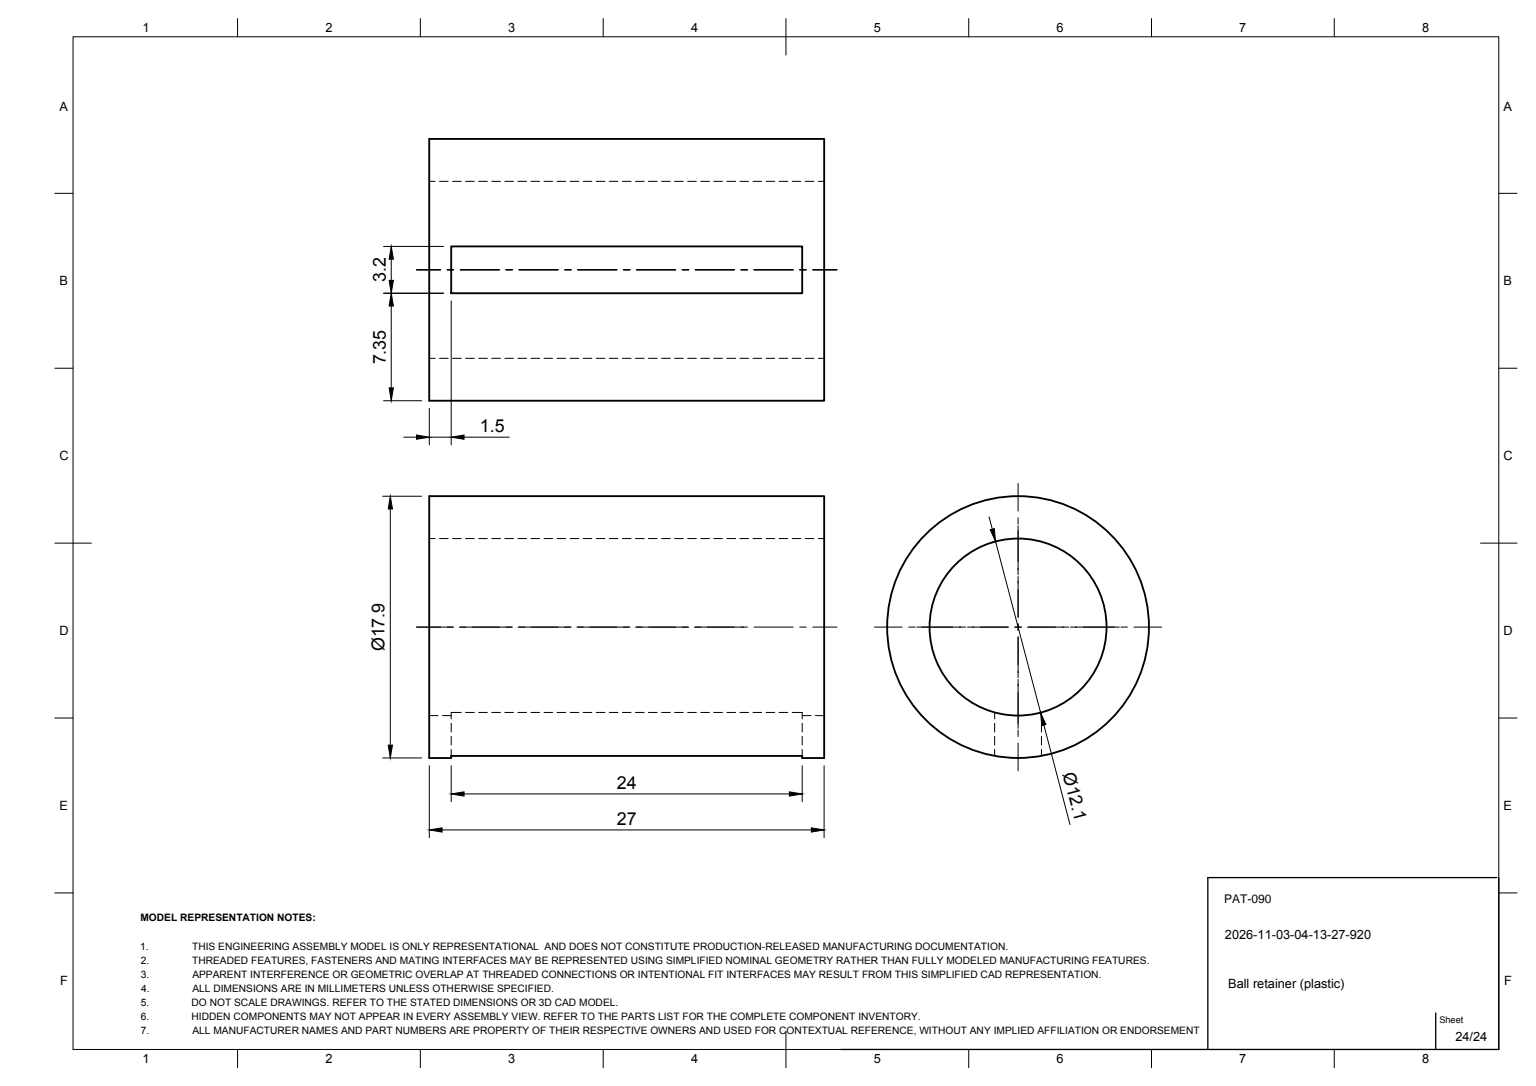
ISO-10303-21;
HEADER;
/* Generated by software containing ST-Developer
 * from STEP Tools, Inc. (www.steptools.com) 
 */

FILE_DESCRIPTION(
/* description */ ('Round-Shaft Linear Stage with Ball Bushings'),
/* implementation_level */ '2;1');

FILE_NAME(
/* name */ 'Ball retainer (plastic).step',
/* time_stamp */ '2026-10-27T10:47:55-07:00',
/* author */ (''),
/* organization */ (''),
/* preprocessor_version */ 'ST-DEVELOPER v20.2',
/* originating_system */ 'Autodesk Translation Framework v15.17.0.0',
/* authorisation */ '');

FILE_SCHEMA (('AUTOMOTIVE_DESIGN { 1 0 10303 214 3 1 1 }'));
ENDSEC;

DATA;
#10=MECHANICAL_DESIGN_GEOMETRIC_PRESENTATION_REPRESENTATION('',(#318),#7835);
#276=SHAPE_REPRESENTATION_RELATIONSHIP('SRR','None',#7966,#297);
#297=ADVANCED_BREP_SHAPE_REPRESENTATION('',(#338),#7830);
#318=STYLED_ITEM('',(#8137),#338);
#338=MANIFOLD_SOLID_BREP('Body1',#4409);
#450=FACE_BOUND('',#1182,.T.);
#451=FACE_BOUND('',#1184,.T.);
#452=FACE_BOUND('',#1186,.T.);
#453=FACE_BOUND('',#1188,.T.);
#575=PLANE('',#5017);
#576=PLANE('',#5020);
#577=PLANE('',#5021);
#578=PLANE('',#5024);
#579=PLANE('',#5025);
#580=PLANE('',#5030);
#810=FACE_OUTER_BOUND('',#1177,.T.);
#811=FACE_OUTER_BOUND('',#1178,.T.);
#812=FACE_OUTER_BOUND('',#1179,.T.);
#813=FACE_OUTER_BOUND('',#1180,.T.);
#814=FACE_OUTER_BOUND('',#1181,.T.);
#815=FACE_OUTER_BOUND('',#1183,.T.);
#816=FACE_OUTER_BOUND('',#1185,.T.);
#817=FACE_OUTER_BOUND('',#1187,.T.);
#1177=EDGE_LOOP('',(#3812,#3813,#3814,#3815));
#1178=EDGE_LOOP('',(#3816,#3817,#3818,#3819));
#1179=EDGE_LOOP('',(#3820,#3821,#3822,#3823));
#1180=EDGE_LOOP('',(#3824,#3825,#3826,#3827));
#1181=EDGE_LOOP('',(#3828));
#1182=EDGE_LOOP('',(#3829));
#1183=EDGE_LOOP('',(#3830,#3831,#3832,#3833));
#1184=EDGE_LOOP('',(#3834,#3835,#3836,#3837));
#1185=EDGE_LOOP('',(#3838));
#1186=EDGE_LOOP('',(#3839));
#1187=EDGE_LOOP('',(#3840,#3841,#3842,#3843));
#1188=EDGE_LOOP('',(#3844,#3845,#3846,#3847));
#1505=LINE('',#7470,#1845);
#1506=LINE('',#7473,#1846);
#1507=LINE('',#7476,#1847);
#1508=LINE('',#7478,#1848);
#1509=LINE('',#7479,#1849);
#1510=LINE('',#7485,#1850);
#1511=LINE('',#7487,#1851);
#1512=LINE('',#7488,#1852);
#1513=LINE('',#7497,#1853);
#1514=LINE('',#7502,#1854);
#1845=VECTOR('',#6172,1.);
#1846=VECTOR('',#6175,1.);
#1847=VECTOR('',#6178,1.);
#1848=VECTOR('',#6179,1.);
#1849=VECTOR('',#6180,1.);
#1850=VECTOR('',#6187,1.);
#1851=VECTOR('',#6190,1.);
#1852=VECTOR('',#6191,1.);
#1853=VECTOR('',#6202,0.895);
#1854=VECTOR('',#6209,0.605);
#2082=CIRCLE('',#5018,0.895);
#2083=CIRCLE('',#5019,0.605);
#2084=CIRCLE('',#5022,0.895);
#2085=CIRCLE('',#5023,0.605);
#2086=CIRCLE('',#5026,0.895);
#2087=CIRCLE('',#5027,0.605);
#2088=CIRCLE('',#5029,0.895);
#2089=CIRCLE('',#5031,0.605);
#2389=VERTEX_POINT('',#7466);
#2390=VERTEX_POINT('',#7467);
#2391=VERTEX_POINT('',#7469);
#2392=VERTEX_POINT('',#7471);
#2393=VERTEX_POINT('',#7475);
#2394=VERTEX_POINT('',#7477);
#2395=VERTEX_POINT('',#7481);
#2396=VERTEX_POINT('',#7483);
#2397=VERTEX_POINT('',#7490);
#2398=VERTEX_POINT('',#7492);
#2399=VERTEX_POINT('',#7495);
#2400=VERTEX_POINT('',#7499);
#2874=EDGE_CURVE('',#2389,#2390,#2082,.T.);
#2875=EDGE_CURVE('',#2391,#2389,#1505,.T.);
#2876=EDGE_CURVE('',#2392,#2391,#2083,.T.);
#2877=EDGE_CURVE('',#2390,#2392,#1506,.T.);
#2878=EDGE_CURVE('',#2390,#2393,#1507,.T.);
#2879=EDGE_CURVE('',#2394,#2392,#1508,.T.);
#2880=EDGE_CURVE('',#2394,#2393,#1509,.T.);
#2881=EDGE_CURVE('',#2393,#2395,#2084,.T.);
#2882=EDGE_CURVE('',#2396,#2394,#2085,.T.);
#2883=EDGE_CURVE('',#2395,#2396,#1510,.T.);
#2884=EDGE_CURVE('',#2395,#2389,#1511,.T.);
#2885=EDGE_CURVE('',#2391,#2396,#1512,.T.);
#2886=EDGE_CURVE('',#2397,#2397,#2086,.T.);
#2887=EDGE_CURVE('',#2398,#2398,#2087,.T.);
#2888=EDGE_CURVE('',#2399,#2399,#2088,.T.);
#2889=EDGE_CURVE('',#2399,#2397,#1513,.T.);
#2890=EDGE_CURVE('',#2400,#2400,#2089,.T.);
#2891=EDGE_CURVE('',#2400,#2398,#1514,.T.);
#3812=ORIENTED_EDGE('',*,*,#2874,.F.);
#3813=ORIENTED_EDGE('',*,*,#2875,.F.);
#3814=ORIENTED_EDGE('',*,*,#2876,.F.);
#3815=ORIENTED_EDGE('',*,*,#2877,.F.);
#3816=ORIENTED_EDGE('',*,*,#2878,.F.);
#3817=ORIENTED_EDGE('',*,*,#2877,.T.);
#3818=ORIENTED_EDGE('',*,*,#2879,.F.);
#3819=ORIENTED_EDGE('',*,*,#2880,.T.);
#3820=ORIENTED_EDGE('',*,*,#2881,.F.);
#3821=ORIENTED_EDGE('',*,*,#2880,.F.);
#3822=ORIENTED_EDGE('',*,*,#2882,.F.);
#3823=ORIENTED_EDGE('',*,*,#2883,.F.);
#3824=ORIENTED_EDGE('',*,*,#2884,.F.);
#3825=ORIENTED_EDGE('',*,*,#2883,.T.);
#3826=ORIENTED_EDGE('',*,*,#2885,.F.);
#3827=ORIENTED_EDGE('',*,*,#2875,.T.);
#3828=ORIENTED_EDGE('',*,*,#2886,.F.);
#3829=ORIENTED_EDGE('',*,*,#2887,.T.);
#3830=ORIENTED_EDGE('',*,*,#2888,.F.);
#3831=ORIENTED_EDGE('',*,*,#2889,.T.);
#3832=ORIENTED_EDGE('',*,*,#2886,.T.);
#3833=ORIENTED_EDGE('',*,*,#2889,.F.);
#3834=ORIENTED_EDGE('',*,*,#2881,.T.);
#3835=ORIENTED_EDGE('',*,*,#2884,.T.);
#3836=ORIENTED_EDGE('',*,*,#2874,.T.);
#3837=ORIENTED_EDGE('',*,*,#2878,.T.);
#3838=ORIENTED_EDGE('',*,*,#2888,.T.);
#3839=ORIENTED_EDGE('',*,*,#2890,.F.);
#3840=ORIENTED_EDGE('',*,*,#2890,.T.);
#3841=ORIENTED_EDGE('',*,*,#2891,.T.);
#3842=ORIENTED_EDGE('',*,*,#2887,.F.);
#3843=ORIENTED_EDGE('',*,*,#2891,.F.);
#3844=ORIENTED_EDGE('',*,*,#2882,.T.);
#3845=ORIENTED_EDGE('',*,*,#2879,.T.);
#3846=ORIENTED_EDGE('',*,*,#2876,.T.);
#3847=ORIENTED_EDGE('',*,*,#2885,.T.);
#4125=CYLINDRICAL_SURFACE('',#5028,0.895);
#4126=CYLINDRICAL_SURFACE('',#5032,0.605);
#4329=ADVANCED_FACE('',(#810),#575,.F.);
#4330=ADVANCED_FACE('',(#811),#576,.F.);
#4331=ADVANCED_FACE('',(#812),#577,.F.);
#4332=ADVANCED_FACE('',(#813),#578,.F.);
#4333=ADVANCED_FACE('',(#814,#450),#579,.T.);
#4334=ADVANCED_FACE('',(#815,#451),#4125,.T.);
#4335=ADVANCED_FACE('',(#816,#452),#580,.T.);
#4336=ADVANCED_FACE('',(#817,#453),#4126,.F.);
#4409=CLOSED_SHELL('',(#4329,#4330,#4331,#4332,#4333,#4334,#4335,#4336));
#5016=AXIS2_PLACEMENT_3D('',#7464,#6166,#6167);
#5017=AXIS2_PLACEMENT_3D('',#7465,#6168,#6169);
#5018=AXIS2_PLACEMENT_3D('',#7468,#6170,#6171);
#5019=AXIS2_PLACEMENT_3D('',#7472,#6173,#6174);
#5020=AXIS2_PLACEMENT_3D('',#7474,#6176,#6177);
#5021=AXIS2_PLACEMENT_3D('',#7480,#6181,#6182);
#5022=AXIS2_PLACEMENT_3D('',#7482,#6183,#6184);
#5023=AXIS2_PLACEMENT_3D('',#7484,#6185,#6186);
#5024=AXIS2_PLACEMENT_3D('',#7486,#6188,#6189);
#5025=AXIS2_PLACEMENT_3D('',#7489,#6192,#6193);
#5026=AXIS2_PLACEMENT_3D('',#7491,#6194,#6195);
#5027=AXIS2_PLACEMENT_3D('',#7493,#6196,#6197);
#5028=AXIS2_PLACEMENT_3D('',#7494,#6198,#6199);
#5029=AXIS2_PLACEMENT_3D('',#7496,#6200,#6201);
#5030=AXIS2_PLACEMENT_3D('',#7498,#6203,#6204);
#5031=AXIS2_PLACEMENT_3D('',#7500,#6205,#6206);
#5032=AXIS2_PLACEMENT_3D('',#7501,#6207,#6208);
#6166=DIRECTION('axis',(0.,0.,1.));
#6167=DIRECTION('refdir',(1.,0.,0.));
#6168=DIRECTION('center_axis',(0.,1.,0.));
#6169=DIRECTION('ref_axis',(0.,0.,1.));
#6170=DIRECTION('center_axis',(0.,1.,0.));
#6171=DIRECTION('ref_axis',(1.,0.,0.));
#6172=DIRECTION('',(1.,0.,0.));
#6173=DIRECTION('center_axis',(0.,-1.,0.));
#6174=DIRECTION('ref_axis',(1.,0.,0.));
#6175=DIRECTION('',(-1.,0.,0.));
#6176=DIRECTION('center_axis',(0.,0.,-1.));
#6177=DIRECTION('ref_axis',(-1.,0.,0.));
#6178=DIRECTION('',(0.,-1.,0.));
#6179=DIRECTION('',(0.,1.,0.));
#6180=DIRECTION('',(1.,0.,0.));
#6181=DIRECTION('center_axis',(0.,-1.,0.));
#6182=DIRECTION('ref_axis',(0.,0.,-1.));
#6183=DIRECTION('center_axis',(0.,-1.,0.));
#6184=DIRECTION('ref_axis',(1.,0.,0.));
#6185=DIRECTION('center_axis',(0.,1.,0.));
#6186=DIRECTION('ref_axis',(1.,0.,0.));
#6187=DIRECTION('',(-1.,0.,0.));
#6188=DIRECTION('center_axis',(0.,0.,1.));
#6189=DIRECTION('ref_axis',(1.,0.,0.));
#6190=DIRECTION('',(0.,1.,0.));
#6191=DIRECTION('',(0.,-1.,0.));
#6192=DIRECTION('center_axis',(0.,1.,0.));
#6193=DIRECTION('ref_axis',(0.,0.,1.));
#6194=DIRECTION('center_axis',(0.,-1.,0.));
#6195=DIRECTION('ref_axis',(1.,0.,0.));
#6196=DIRECTION('center_axis',(0.,-1.,0.));
#6197=DIRECTION('ref_axis',(1.,0.,0.));
#6198=DIRECTION('center_axis',(0.,-1.,0.));
#6199=DIRECTION('ref_axis',(1.,0.,0.));
#6200=DIRECTION('center_axis',(0.,-1.,0.));
#6201=DIRECTION('ref_axis',(1.,0.,0.));
#6202=DIRECTION('',(0.,1.,0.));
#6203=DIRECTION('center_axis',(0.,-1.,0.));
#6204=DIRECTION('ref_axis',(0.,0.,-1.));
#6205=DIRECTION('center_axis',(0.,-1.,0.));
#6206=DIRECTION('ref_axis',(1.,0.,0.));
#6207=DIRECTION('center_axis',(0.,-1.,0.));
#6208=DIRECTION('ref_axis',(1.,0.,0.));
#6209=DIRECTION('',(0.,1.,0.));
#7464=CARTESIAN_POINT('',(0.,0.,0.));
#7465=CARTESIAN_POINT('Origin',(0.75,1.2,0.));
#7466=CARTESIAN_POINT('',(0.880582193778639,1.2,0.16));
#7467=CARTESIAN_POINT('',(0.880582193778639,1.2,-0.16));
#7468=CARTESIAN_POINT('Origin',(0.,1.2,0.));
#7469=CARTESIAN_POINT('',(0.583459510163302,1.2,0.16));
#7470=CARTESIAN_POINT('',(0.57,1.2,0.16));
#7471=CARTESIAN_POINT('',(0.583459510163302,1.2,-0.16));
#7472=CARTESIAN_POINT('Origin',(0.,1.2,0.));
#7473=CARTESIAN_POINT('',(0.93,1.2,-0.16));
#7474=CARTESIAN_POINT('Origin',(0.93,0.,-0.16));
#7475=CARTESIAN_POINT('',(0.880582193778639,-1.2,-0.16));
#7476=CARTESIAN_POINT('',(0.880582193778639,0.,-0.16));
#7477=CARTESIAN_POINT('',(0.583459510163302,-1.2,-0.16));
#7478=CARTESIAN_POINT('',(0.583459510163302,0.,-0.16));
#7479=CARTESIAN_POINT('',(0.93,-1.2,-0.16));
#7480=CARTESIAN_POINT('Origin',(0.75,-1.2,0.));
#7481=CARTESIAN_POINT('',(0.880582193778639,-1.2,0.16));
#7482=CARTESIAN_POINT('Origin',(0.,-1.2,0.));
#7483=CARTESIAN_POINT('',(0.583459510163302,-1.2,0.16));
#7484=CARTESIAN_POINT('Origin',(0.,-1.2,0.));
#7485=CARTESIAN_POINT('',(0.57,-1.2,0.16));
#7486=CARTESIAN_POINT('Origin',(0.57,0.,0.16));
#7487=CARTESIAN_POINT('',(0.880582193778639,0.,0.16));
#7488=CARTESIAN_POINT('',(0.583459510163302,0.,0.16));
#7489=CARTESIAN_POINT('Origin',(0.895,1.35,0.));
#7490=CARTESIAN_POINT('',(-0.895,1.35,-1.09605888523688E-16));
#7491=CARTESIAN_POINT('Origin',(0.,1.35,0.));
#7492=CARTESIAN_POINT('',(-0.605,1.35,-7.40911313484149E-17));
#7493=CARTESIAN_POINT('Origin',(0.,1.35,0.));
#7494=CARTESIAN_POINT('Origin',(0.,0.,0.));
#7495=CARTESIAN_POINT('',(-0.895,-1.35,-1.09605888523688E-16));
#7496=CARTESIAN_POINT('Origin',(0.,-1.35,0.));
#7497=CARTESIAN_POINT('',(-0.895,0.,-1.09605888523688E-16));
#7498=CARTESIAN_POINT('Origin',(0.605,-1.35,0.));
#7499=CARTESIAN_POINT('',(-0.605,-1.35,-7.40911313484149E-17));
#7500=CARTESIAN_POINT('Origin',(0.,-1.35,0.));
#7501=CARTESIAN_POINT('Origin',(0.,0.,0.));
#7502=CARTESIAN_POINT('',(-0.605,0.,-7.40911313484149E-17));
#7804=UNCERTAINTY_MEASURE_WITH_UNIT(LENGTH_MEASURE(0.001),#7836,
'DISTANCE_ACCURACY_VALUE',
'Maximum model space distance between geometric entities at asserted c
onnectivities');
#7809=UNCERTAINTY_MEASURE_WITH_UNIT(LENGTH_MEASURE(0.001),#7836,
'DISTANCE_ACCURACY_VALUE',
'Maximum model space distance between geometric entities at asserted c
onnectivities');
#7830=(
GEOMETRIC_REPRESENTATION_CONTEXT(3)
GLOBAL_UNCERTAINTY_ASSIGNED_CONTEXT((#7804))
GLOBAL_UNIT_ASSIGNED_CONTEXT((#7836,#7838,#7839))
REPRESENTATION_CONTEXT('','3D')
);
#7835=(
GEOMETRIC_REPRESENTATION_CONTEXT(3)
GLOBAL_UNCERTAINTY_ASSIGNED_CONTEXT((#7809))
GLOBAL_UNIT_ASSIGNED_CONTEXT((#7836,#7838,#7839))
REPRESENTATION_CONTEXT('','3D')
);
#7836=(
LENGTH_UNIT()
NAMED_UNIT(*)
SI_UNIT(.CENTI.,.METRE.)
);
#7838=(
NAMED_UNIT(*)
PLANE_ANGLE_UNIT()
SI_UNIT($,.RADIAN.)
);
#7839=(
NAMED_UNIT(*)
SI_UNIT($,.STERADIAN.)
SOLID_ANGLE_UNIT()
);
#7860=SHAPE_DEFINITION_REPRESENTATION(#7885,#7966);
#7885=PRODUCT_DEFINITION_SHAPE('',$,#7992);
#7966=SHAPE_REPRESENTATION('',(#5016),#7830);
#7971=PRODUCT_DEFINITION_CONTEXT('part definition',#8048,'design');
#7992=PRODUCT_DEFINITION('Ball retainer (plastic)',
'Ball retainer (plastic)',#8017,#7971);
#8017=PRODUCT_DEFINITION_FORMATION('',$,#8070);
#8048=APPLICATION_CONTEXT(
'Core Data for Automotive Mechanical Design Process');
#8049=PRODUCT_CONTEXT('part definition',#8048,'mechanical');
#8070=PRODUCT('Ball retainer (plastic)','Ball retainer (plastic)',
'Ball retainer (plastic)',(#8049));
#8131=COLOUR_RGB('Sky Blue',0.24,0.69,0.87);
#8132=FILL_AREA_STYLE_COLOUR('',#8131);
#8133=FILL_AREA_STYLE('',(#8132));
#8134=SURFACE_STYLE_FILL_AREA(#8133);
#8135=SURFACE_SIDE_STYLE('',(#8134));
#8136=SURFACE_STYLE_USAGE(.BOTH.,#8135);
#8137=PRESENTATION_STYLE_ASSIGNMENT((#8136));
ENDSEC;
END-ISO-10303-21;
